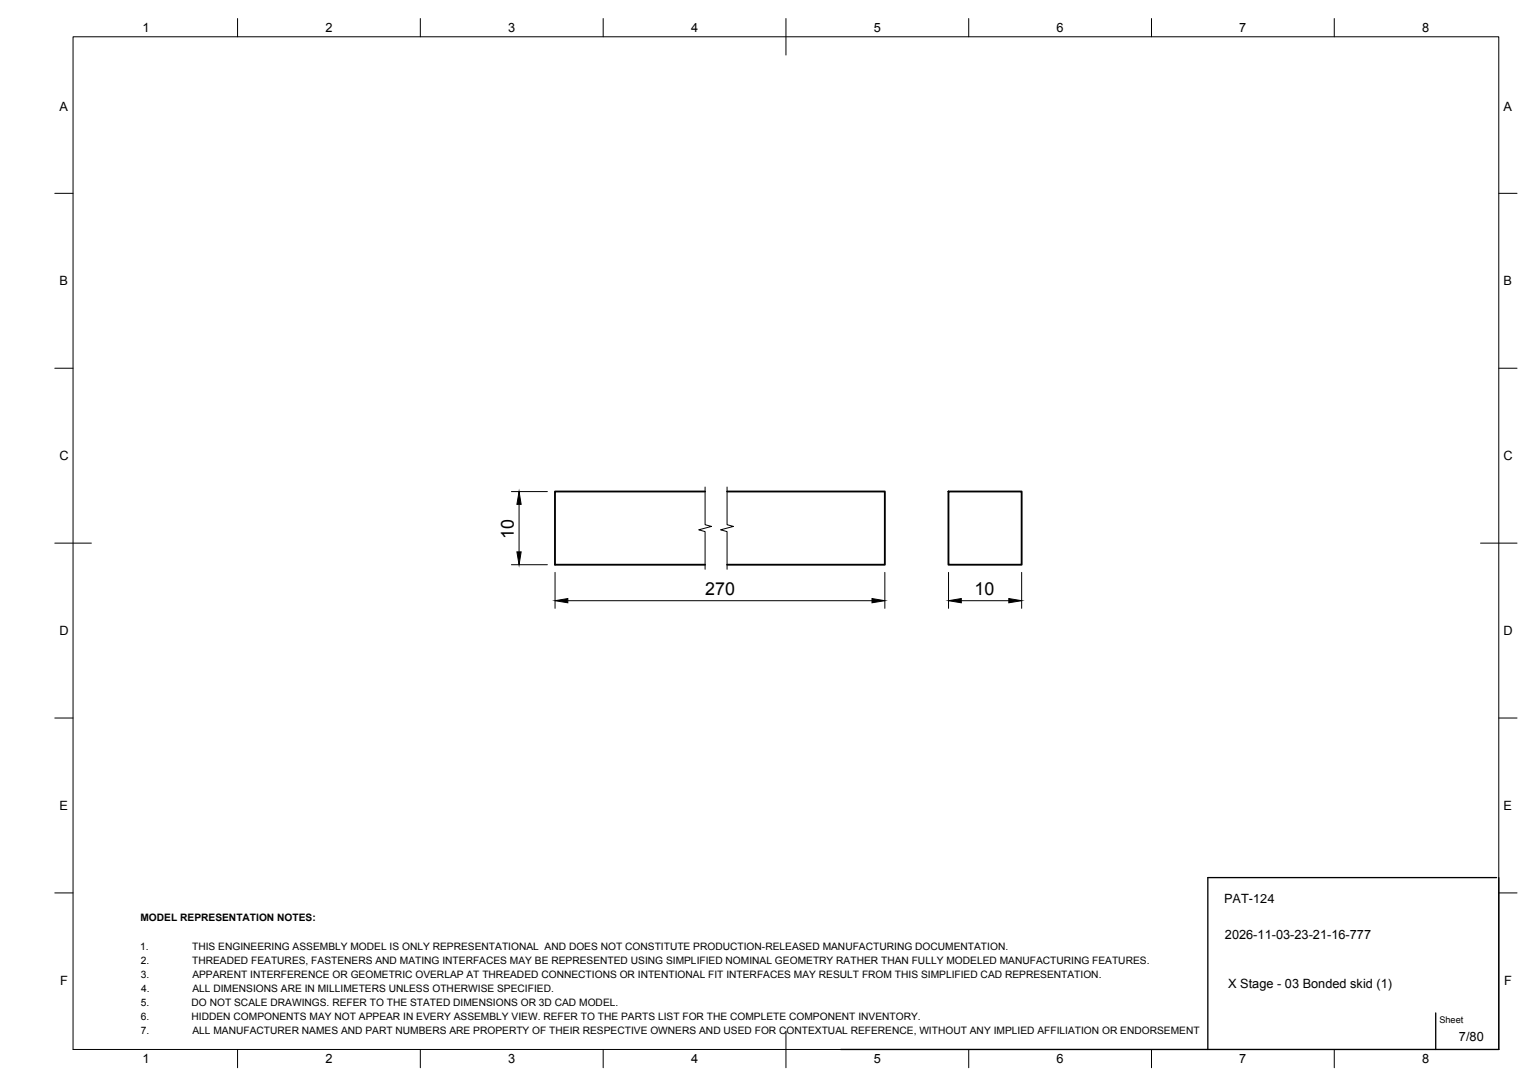
ISO-10303-21;
HEADER;
/* Generated by software containing ST-Developer
 * from STEP Tools, Inc. (www.steptools.com) 
 */

FILE_DESCRIPTION(
/* description */ ('XY cross-slide table'),
/* implementation_level */ '2;1');

FILE_NAME(
/* name */ 'X Stage - 03 Bonded skid (1).step',
/* time_stamp */ '2026-10-28T03:22:46-07:00',
/* author */ (''),
/* organization */ (''),
/* preprocessor_version */ 'ST-DEVELOPER v20.2',
/* originating_system */ 'Autodesk Translation Framework v15.17.0.0',
/* authorisation */ '');

FILE_SCHEMA (('AUTOMOTIVE_DESIGN { 1 0 10303 214 3 1 1 }'));
ENDSEC;

DATA;
#10=MECHANICAL_DESIGN_GEOMETRIC_PRESENTATION_REPRESENTATION('',(#1672),#62984);
#1506=SHAPE_REPRESENTATION_RELATIONSHIP('SRR','None',#63354,#1589);
#1589=ADVANCED_BREP_SHAPE_REPRESENTATION('',(#1785),#62891);
#1672=STYLED_ITEM('',(#63898),#1785);
#1785=MANIFOLD_SOLID_BREP('Body1',#22966);
#2308=PLANE('',#24048);
#2309=PLANE('',#24049);
#2310=PLANE('',#24050);
#2311=PLANE('',#24051);
#2312=PLANE('',#24052);
#2313=PLANE('',#24053);
#2891=FACE_OUTER_BOUND('',#4225,.T.);
#2892=FACE_OUTER_BOUND('',#4226,.T.);
#2893=FACE_OUTER_BOUND('',#4227,.T.);
#2894=FACE_OUTER_BOUND('',#4228,.T.);
#2895=FACE_OUTER_BOUND('',#4229,.T.);
#2896=FACE_OUTER_BOUND('',#4230,.T.);
#4225=EDGE_LOOP('',(#15012,#15013,#15014,#15015));
#4226=EDGE_LOOP('',(#15016,#15017,#15018,#15019));
#4227=EDGE_LOOP('',(#15020,#15021,#15022,#15023));
#4228=EDGE_LOOP('',(#15024,#15025,#15026,#15027));
#4229=EDGE_LOOP('',(#15028,#15029,#15030,#15031));
#4230=EDGE_LOOP('',(#15032,#15033,#15034,#15035));
#5940=LINE('',#32991,#7427);
#5941=LINE('',#32993,#7428);
#5942=LINE('',#32995,#7429);
#5943=LINE('',#32996,#7430);
#5944=LINE('',#32999,#7431);
#5945=LINE('',#33001,#7432);
#5946=LINE('',#33002,#7433);
#5947=LINE('',#33005,#7434);
#5948=LINE('',#33007,#7435);
#5949=LINE('',#33008,#7436);
#5950=LINE('',#33010,#7437);
#5951=LINE('',#33011,#7438);
#7427=VECTOR('',#26593,1.);
#7428=VECTOR('',#26594,1.);
#7429=VECTOR('',#26595,1.);
#7430=VECTOR('',#26596,1.);
#7431=VECTOR('',#26599,1.);
#7432=VECTOR('',#26600,1.);
#7433=VECTOR('',#26601,1.);
#7434=VECTOR('',#26604,1.);
#7435=VECTOR('',#26605,1.);
#7436=VECTOR('',#26606,1.);
#7437=VECTOR('',#26609,1.);
#7438=VECTOR('',#26610,1.);
#9809=VERTEX_POINT('',#32989);
#9810=VERTEX_POINT('',#32990);
#9811=VERTEX_POINT('',#32992);
#9812=VERTEX_POINT('',#32994);
#9813=VERTEX_POINT('',#32998);
#9814=VERTEX_POINT('',#33000);
#9815=VERTEX_POINT('',#33004);
#9816=VERTEX_POINT('',#33006);
#11890=EDGE_CURVE('',#9809,#9810,#5940,.T.);
#11891=EDGE_CURVE('',#9810,#9811,#5941,.T.);
#11892=EDGE_CURVE('',#9812,#9811,#5942,.T.);
#11893=EDGE_CURVE('',#9809,#9812,#5943,.T.);
#11894=EDGE_CURVE('',#9813,#9809,#5944,.T.);
#11895=EDGE_CURVE('',#9814,#9812,#5945,.T.);
#11896=EDGE_CURVE('',#9813,#9814,#5946,.T.);
#11897=EDGE_CURVE('',#9815,#9813,#5947,.T.);
#11898=EDGE_CURVE('',#9816,#9814,#5948,.T.);
#11899=EDGE_CURVE('',#9815,#9816,#5949,.T.);
#11900=EDGE_CURVE('',#9810,#9815,#5950,.T.);
#11901=EDGE_CURVE('',#9811,#9816,#5951,.T.);
#15012=ORIENTED_EDGE('',*,*,#11890,.T.);
#15013=ORIENTED_EDGE('',*,*,#11891,.T.);
#15014=ORIENTED_EDGE('',*,*,#11892,.F.);
#15015=ORIENTED_EDGE('',*,*,#11893,.F.);
#15016=ORIENTED_EDGE('',*,*,#11894,.T.);
#15017=ORIENTED_EDGE('',*,*,#11893,.T.);
#15018=ORIENTED_EDGE('',*,*,#11895,.F.);
#15019=ORIENTED_EDGE('',*,*,#11896,.F.);
#15020=ORIENTED_EDGE('',*,*,#11897,.T.);
#15021=ORIENTED_EDGE('',*,*,#11896,.T.);
#15022=ORIENTED_EDGE('',*,*,#11898,.F.);
#15023=ORIENTED_EDGE('',*,*,#11899,.F.);
#15024=ORIENTED_EDGE('',*,*,#11900,.T.);
#15025=ORIENTED_EDGE('',*,*,#11899,.T.);
#15026=ORIENTED_EDGE('',*,*,#11901,.F.);
#15027=ORIENTED_EDGE('',*,*,#11891,.F.);
#15028=ORIENTED_EDGE('',*,*,#11901,.T.);
#15029=ORIENTED_EDGE('',*,*,#11898,.T.);
#15030=ORIENTED_EDGE('',*,*,#11895,.T.);
#15031=ORIENTED_EDGE('',*,*,#11892,.T.);
#15032=ORIENTED_EDGE('',*,*,#11900,.F.);
#15033=ORIENTED_EDGE('',*,*,#11890,.F.);
#15034=ORIENTED_EDGE('',*,*,#11894,.F.);
#15035=ORIENTED_EDGE('',*,*,#11897,.F.);
#21672=ADVANCED_FACE('',(#2891),#2308,.T.);
#21673=ADVANCED_FACE('',(#2892),#2309,.T.);
#21674=ADVANCED_FACE('',(#2893),#2310,.T.);
#21675=ADVANCED_FACE('',(#2894),#2311,.T.);
#21676=ADVANCED_FACE('',(#2895),#2312,.T.);
#21677=ADVANCED_FACE('',(#2896),#2313,.F.);
#22966=CLOSED_SHELL('',(#21672,#21673,#21674,#21675,#21676,#21677));
#24047=AXIS2_PLACEMENT_3D('',#32987,#26589,#26590);
#24048=AXIS2_PLACEMENT_3D('',#32988,#26591,#26592);
#24049=AXIS2_PLACEMENT_3D('',#32997,#26597,#26598);
#24050=AXIS2_PLACEMENT_3D('',#33003,#26602,#26603);
#24051=AXIS2_PLACEMENT_3D('',#33009,#26607,#26608);
#24052=AXIS2_PLACEMENT_3D('',#33012,#26611,#26612);
#24053=AXIS2_PLACEMENT_3D('',#33013,#26613,#26614);
#26589=DIRECTION('axis',(0.,0.,1.));
#26590=DIRECTION('refdir',(1.,0.,0.));
#26591=DIRECTION('center_axis',(0.,1.,0.));
#26592=DIRECTION('ref_axis',(-1.,0.,0.));
#26593=DIRECTION('',(-1.,0.,0.));
#26594=DIRECTION('',(0.,0.,1.));
#26595=DIRECTION('',(-1.,0.,0.));
#26596=DIRECTION('',(0.,0.,1.));
#26597=DIRECTION('center_axis',(1.,0.,0.));
#26598=DIRECTION('ref_axis',(0.,1.,0.));
#26599=DIRECTION('',(0.,1.,0.));
#26600=DIRECTION('',(0.,1.,0.));
#26601=DIRECTION('',(0.,0.,1.));
#26602=DIRECTION('center_axis',(0.,-1.,0.));
#26603=DIRECTION('ref_axis',(1.,0.,0.));
#26604=DIRECTION('',(1.,0.,0.));
#26605=DIRECTION('',(1.,0.,0.));
#26606=DIRECTION('',(0.,0.,1.));
#26607=DIRECTION('center_axis',(-1.,0.,0.));
#26608=DIRECTION('ref_axis',(0.,-1.,0.));
#26609=DIRECTION('',(0.,-1.,0.));
#26610=DIRECTION('',(0.,-1.,0.));
#26611=DIRECTION('center_axis',(0.,0.,1.));
#26612=DIRECTION('ref_axis',(1.,0.,0.));
#26613=DIRECTION('center_axis',(0.,0.,1.));
#26614=DIRECTION('ref_axis',(1.,0.,0.));
#32987=CARTESIAN_POINT('',(0.,0.,0.));
#32988=CARTESIAN_POINT('Origin',(27.,5.,-1.));
#32989=CARTESIAN_POINT('',(27.,5.,-1.));
#32990=CARTESIAN_POINT('',(0.,5.,-1.));
#32991=CARTESIAN_POINT('',(27.,5.,-1.));
#32992=CARTESIAN_POINT('',(0.,5.,0.));
#32993=CARTESIAN_POINT('',(0.,5.,-1.));
#32994=CARTESIAN_POINT('',(27.,5.,0.));
#32995=CARTESIAN_POINT('',(27.,5.,0.));
#32996=CARTESIAN_POINT('',(27.,5.,-1.));
#32997=CARTESIAN_POINT('Origin',(27.,4.,-1.));
#32998=CARTESIAN_POINT('',(27.,4.,-1.));
#32999=CARTESIAN_POINT('',(27.,4.,-1.));
#33000=CARTESIAN_POINT('',(27.,4.,0.));
#33001=CARTESIAN_POINT('',(27.,4.,0.));
#33002=CARTESIAN_POINT('',(27.,4.,-1.));
#33003=CARTESIAN_POINT('Origin',(0.,4.,-1.));
#33004=CARTESIAN_POINT('',(0.,4.,-1.));
#33005=CARTESIAN_POINT('',(0.,4.,-1.));
#33006=CARTESIAN_POINT('',(0.,4.,0.));
#33007=CARTESIAN_POINT('',(0.,4.,0.));
#33008=CARTESIAN_POINT('',(0.,4.,-1.));
#33009=CARTESIAN_POINT('Origin',(0.,5.,-1.));
#33010=CARTESIAN_POINT('',(0.,5.,-1.));
#33011=CARTESIAN_POINT('',(0.,5.,0.));
#33012=CARTESIAN_POINT('Origin',(13.5,4.5,0.));
#33013=CARTESIAN_POINT('Origin',(13.5,4.5,-1.));
#62792=UNCERTAINTY_MEASURE_WITH_UNIT(LENGTH_MEASURE(0.001),#62985,
'DISTANCE_ACCURACY_VALUE',
'Maximum model space distance between geometric entities at asserted c
onnectivities');
#62885=UNCERTAINTY_MEASURE_WITH_UNIT(LENGTH_MEASURE(0.001),#62985,
'DISTANCE_ACCURACY_VALUE',
'Maximum model space distance between geometric entities at asserted c
onnectivities');
#62891=(
GEOMETRIC_REPRESENTATION_CONTEXT(3)
GLOBAL_UNCERTAINTY_ASSIGNED_CONTEXT((#62792))
GLOBAL_UNIT_ASSIGNED_CONTEXT((#62985,#62987,#62988))
REPRESENTATION_CONTEXT('','3D')
);
#62984=(
GEOMETRIC_REPRESENTATION_CONTEXT(3)
GLOBAL_UNCERTAINTY_ASSIGNED_CONTEXT((#62885))
GLOBAL_UNIT_ASSIGNED_CONTEXT((#62985,#62987,#62988))
REPRESENTATION_CONTEXT('','3D')
);
#62985=(
LENGTH_UNIT()
NAMED_UNIT(*)
SI_UNIT(.CENTI.,.METRE.)
);
#62987=(
NAMED_UNIT(*)
PLANE_ANGLE_UNIT()
SI_UNIT($,.RADIAN.)
);
#62988=(
NAMED_UNIT(*)
SI_UNIT($,.STERADIAN.)
SOLID_ANGLE_UNIT()
);
#62994=SHAPE_DEFINITION_REPRESENTATION(#63092,#63354);
#63092=PRODUCT_DEFINITION_SHAPE('',$,#63453);
#63354=SHAPE_REPRESENTATION('',(#24047),#62891);
#63447=PRODUCT_DEFINITION_CONTEXT('part definition',#63743,'design');
#63453=PRODUCT_DEFINITION('X Stage - 03 Bonded skid (1)',
'X Stage - 03 Bonded skid (1)',#63551,#63447);
#63551=PRODUCT_DEFINITION_FORMATION('',$,#63750);
#63743=APPLICATION_CONTEXT(
'Core Data for Automotive Mechanical Design Process');
#63744=PRODUCT_CONTEXT('part definition',#63743,'mechanical');
#63750=PRODUCT('X Stage - 03 Bonded skid (1)',
'X Stage - 03 Bonded skid (1)','X Stage - 03 Bonded skid (1)',(#63744));
#63892=COLOUR_RGB('Light Blue',0.38,0.62,0.78);
#63893=FILL_AREA_STYLE_COLOUR('',#63892);
#63894=FILL_AREA_STYLE('',(#63893));
#63895=SURFACE_STYLE_FILL_AREA(#63894);
#63896=SURFACE_SIDE_STYLE('',(#63895));
#63897=SURFACE_STYLE_USAGE(.BOTH.,#63896);
#63898=PRESENTATION_STYLE_ASSIGNMENT((#63897));
ENDSEC;
END-ISO-10303-21;
